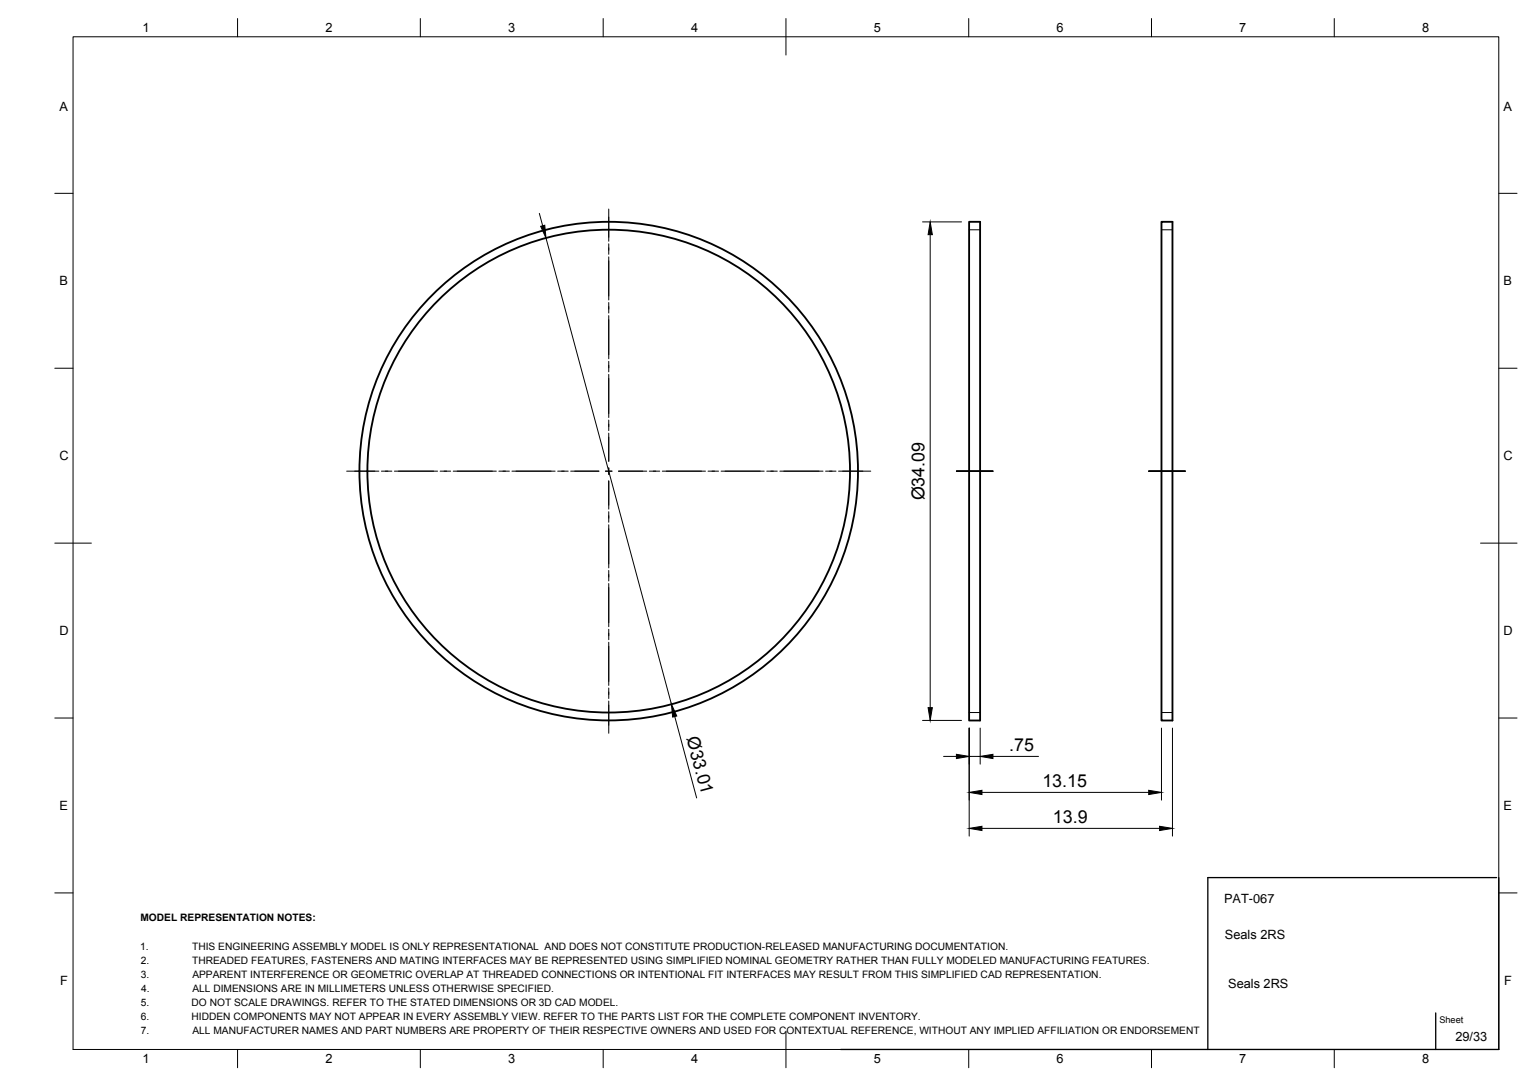
ISO-10303-21;
HEADER;
/* Generated by software containing ST-Developer
 * from STEP Tools, Inc. (www.steptools.com) 
 */

FILE_DESCRIPTION(
/* description */ ('Lifting hook block with sheave'),
/* implementation_level */ '2;1');

FILE_NAME(
/* name */ 'Seals 2RS.step',
/* time_stamp */ '2026-10-28T03:23:54-07:00',
/* author */ (''),
/* organization */ (''),
/* preprocessor_version */ 'ST-DEVELOPER v20.2',
/* originating_system */ 'Autodesk Translation Framework v15.17.0.0',
/* authorisation */ '');

FILE_SCHEMA (('AUTOMOTIVE_DESIGN { 1 0 10303 214 3 1 1 }'));
ENDSEC;

DATA;
#10=MECHANICAL_DESIGN_GEOMETRIC_PRESENTATION_REPRESENTATION('',(#382,#383),#9391);
#315=SHAPE_REPRESENTATION_RELATIONSHIP('SRR','None',#9548,#345);
#345=ADVANCED_BREP_SHAPE_REPRESENTATION('',(#418,#419),#9383);
#382=STYLED_ITEM('',(#9759),#418);
#383=STYLED_ITEM('',(#9759),#419);
#418=MANIFOLD_SOLID_BREP('Body1',#4920);
#419=MANIFOLD_SOLID_BREP('Body2',#4921);
#638=LINE('',#9043,#926);
#639=LINE('',#9048,#927);
#640=LINE('',#9057,#928);
#641=LINE('',#9062,#929);
#926=VECTOR('',#7225,1.70469);
#927=VECTOR('',#7232,1.65031);
#928=VECTOR('',#7243,1.70469);
#929=VECTOR('',#7250,1.65031);
#1089=CYLINDRICAL_SURFACE('',#5798,1.70469);
#1090=CYLINDRICAL_SURFACE('',#5802,1.65031);
#1091=CYLINDRICAL_SURFACE('',#5806,1.70469);
#1092=CYLINDRICAL_SURFACE('',#5810,1.65031);
#1207=FACE_BOUND('',#1842,.T.);
#1208=FACE_BOUND('',#1845,.T.);
#1209=FACE_BOUND('',#1848,.T.);
#1210=FACE_BOUND('',#1851,.T.);
#1452=FACE_OUTER_BOUND('',#1841,.T.);
#1453=FACE_OUTER_BOUND('',#1843,.T.);
#1454=FACE_OUTER_BOUND('',#1844,.T.);
#1455=FACE_OUTER_BOUND('',#1846,.T.);
#1456=FACE_OUTER_BOUND('',#1847,.T.);
#1457=FACE_OUTER_BOUND('',#1849,.T.);
#1458=FACE_OUTER_BOUND('',#1850,.T.);
#1459=FACE_OUTER_BOUND('',#1852,.T.);
#1841=EDGE_LOOP('',(#4222));
#1842=EDGE_LOOP('',(#4223));
#1843=EDGE_LOOP('',(#4224,#4225,#4226,#4227));
#1844=EDGE_LOOP('',(#4228));
#1845=EDGE_LOOP('',(#4229));
#1846=EDGE_LOOP('',(#4230,#4231,#4232,#4233));
#1847=EDGE_LOOP('',(#4234));
#1848=EDGE_LOOP('',(#4235));
#1849=EDGE_LOOP('',(#4236,#4237,#4238,#4239));
#1850=EDGE_LOOP('',(#4240));
#1851=EDGE_LOOP('',(#4241));
#1852=EDGE_LOOP('',(#4242,#4243,#4244,#4245));
#2167=CIRCLE('',#5796,1.70469);
#2168=CIRCLE('',#5797,1.65031);
#2169=CIRCLE('',#5799,1.70469);
#2170=CIRCLE('',#5801,1.65031);
#2171=CIRCLE('',#5804,1.70469);
#2172=CIRCLE('',#5805,1.65031);
#2173=CIRCLE('',#5807,1.70469);
#2174=CIRCLE('',#5809,1.65031);
#2544=VERTEX_POINT('',#9036);
#2545=VERTEX_POINT('',#9038);
#2546=VERTEX_POINT('',#9041);
#2547=VERTEX_POINT('',#9045);
#2548=VERTEX_POINT('',#9050);
#2549=VERTEX_POINT('',#9052);
#2550=VERTEX_POINT('',#9055);
#2551=VERTEX_POINT('',#9059);
#3115=EDGE_CURVE('',#2544,#2544,#2167,.T.);
#3116=EDGE_CURVE('',#2545,#2545,#2168,.T.);
#3117=EDGE_CURVE('',#2546,#2546,#2169,.T.);
#3118=EDGE_CURVE('',#2546,#2544,#638,.T.);
#3119=EDGE_CURVE('',#2547,#2547,#2170,.T.);
#3120=EDGE_CURVE('',#2547,#2545,#639,.T.);
#3121=EDGE_CURVE('',#2548,#2548,#2171,.T.);
#3122=EDGE_CURVE('',#2549,#2549,#2172,.T.);
#3123=EDGE_CURVE('',#2550,#2550,#2173,.T.);
#3124=EDGE_CURVE('',#2550,#2548,#640,.T.);
#3125=EDGE_CURVE('',#2551,#2551,#2174,.T.);
#3126=EDGE_CURVE('',#2551,#2549,#641,.T.);
#4222=ORIENTED_EDGE('',*,*,#3115,.F.);
#4223=ORIENTED_EDGE('',*,*,#3116,.T.);
#4224=ORIENTED_EDGE('',*,*,#3117,.F.);
#4225=ORIENTED_EDGE('',*,*,#3118,.T.);
#4226=ORIENTED_EDGE('',*,*,#3115,.T.);
#4227=ORIENTED_EDGE('',*,*,#3118,.F.);
#4228=ORIENTED_EDGE('',*,*,#3117,.T.);
#4229=ORIENTED_EDGE('',*,*,#3119,.F.);
#4230=ORIENTED_EDGE('',*,*,#3119,.T.);
#4231=ORIENTED_EDGE('',*,*,#3120,.T.);
#4232=ORIENTED_EDGE('',*,*,#3116,.F.);
#4233=ORIENTED_EDGE('',*,*,#3120,.F.);
#4234=ORIENTED_EDGE('',*,*,#3121,.F.);
#4235=ORIENTED_EDGE('',*,*,#3122,.T.);
#4236=ORIENTED_EDGE('',*,*,#3123,.F.);
#4237=ORIENTED_EDGE('',*,*,#3124,.T.);
#4238=ORIENTED_EDGE('',*,*,#3121,.T.);
#4239=ORIENTED_EDGE('',*,*,#3124,.F.);
#4240=ORIENTED_EDGE('',*,*,#3123,.T.);
#4241=ORIENTED_EDGE('',*,*,#3125,.F.);
#4242=ORIENTED_EDGE('',*,*,#3125,.T.);
#4243=ORIENTED_EDGE('',*,*,#3126,.T.);
#4244=ORIENTED_EDGE('',*,*,#3122,.F.);
#4245=ORIENTED_EDGE('',*,*,#3126,.F.);
#4560=PLANE('',#5795);
#4561=PLANE('',#5800);
#4562=PLANE('',#5803);
#4563=PLANE('',#5808);
#4828=ADVANCED_FACE('',(#1452,#1207),#4560,.T.);
#4829=ADVANCED_FACE('',(#1453),#1089,.T.);
#4830=ADVANCED_FACE('',(#1454,#1208),#4561,.T.);
#4831=ADVANCED_FACE('',(#1455),#1090,.F.);
#4832=ADVANCED_FACE('',(#1456,#1209),#4562,.T.);
#4833=ADVANCED_FACE('',(#1457),#1091,.T.);
#4834=ADVANCED_FACE('',(#1458,#1210),#4563,.T.);
#4835=ADVANCED_FACE('',(#1459),#1092,.F.);
#4920=CLOSED_SHELL('',(#4828,#4829,#4830,#4831));
#4921=CLOSED_SHELL('',(#4832,#4833,#4834,#4835));
#5794=AXIS2_PLACEMENT_3D('',#9034,#7213,#7214);
#5795=AXIS2_PLACEMENT_3D('',#9035,#7215,#7216);
#5796=AXIS2_PLACEMENT_3D('',#9037,#7217,#7218);
#5797=AXIS2_PLACEMENT_3D('',#9039,#7219,#7220);
#5798=AXIS2_PLACEMENT_3D('',#9040,#7221,#7222);
#5799=AXIS2_PLACEMENT_3D('',#9042,#7223,#7224);
#5800=AXIS2_PLACEMENT_3D('',#9044,#7226,#7227);
#5801=AXIS2_PLACEMENT_3D('',#9046,#7228,#7229);
#5802=AXIS2_PLACEMENT_3D('',#9047,#7230,#7231);
#5803=AXIS2_PLACEMENT_3D('',#9049,#7233,#7234);
#5804=AXIS2_PLACEMENT_3D('',#9051,#7235,#7236);
#5805=AXIS2_PLACEMENT_3D('',#9053,#7237,#7238);
#5806=AXIS2_PLACEMENT_3D('',#9054,#7239,#7240);
#5807=AXIS2_PLACEMENT_3D('',#9056,#7241,#7242);
#5808=AXIS2_PLACEMENT_3D('',#9058,#7244,#7245);
#5809=AXIS2_PLACEMENT_3D('',#9060,#7246,#7247);
#5810=AXIS2_PLACEMENT_3D('',#9061,#7248,#7249);
#7213=DIRECTION('axis',(0.,0.,1.));
#7214=DIRECTION('refdir',(1.,0.,0.));
#7215=DIRECTION('center_axis',(0.,1.,0.));
#7216=DIRECTION('ref_axis',(0.,0.,1.));
#7217=DIRECTION('center_axis',(0.,-1.,0.));
#7218=DIRECTION('ref_axis',(1.,0.,0.));
#7219=DIRECTION('center_axis',(0.,-1.,0.));
#7220=DIRECTION('ref_axis',(1.,0.,0.));
#7221=DIRECTION('center_axis',(0.,-1.,0.));
#7222=DIRECTION('ref_axis',(1.,0.,0.));
#7223=DIRECTION('center_axis',(0.,-1.,0.));
#7224=DIRECTION('ref_axis',(1.,0.,0.));
#7225=DIRECTION('',(0.,1.,0.));
#7226=DIRECTION('center_axis',(0.,-1.,0.));
#7227=DIRECTION('ref_axis',(0.,0.,-1.));
#7228=DIRECTION('center_axis',(0.,-1.,0.));
#7229=DIRECTION('ref_axis',(1.,0.,0.));
#7230=DIRECTION('center_axis',(0.,-1.,0.));
#7231=DIRECTION('ref_axis',(1.,0.,0.));
#7232=DIRECTION('',(0.,1.,0.));
#7233=DIRECTION('center_axis',(0.,1.,0.));
#7234=DIRECTION('ref_axis',(0.,0.,1.));
#7235=DIRECTION('center_axis',(0.,-1.,0.));
#7236=DIRECTION('ref_axis',(1.,0.,0.));
#7237=DIRECTION('center_axis',(0.,-1.,0.));
#7238=DIRECTION('ref_axis',(1.,0.,0.));
#7239=DIRECTION('center_axis',(0.,-1.,0.));
#7240=DIRECTION('ref_axis',(1.,0.,0.));
#7241=DIRECTION('center_axis',(0.,-1.,0.));
#7242=DIRECTION('ref_axis',(1.,0.,0.));
#7243=DIRECTION('',(0.,1.,0.));
#7244=DIRECTION('center_axis',(0.,-1.,0.));
#7245=DIRECTION('ref_axis',(0.,0.,-1.));
#7246=DIRECTION('center_axis',(0.,-1.,0.));
#7247=DIRECTION('ref_axis',(1.,0.,0.));
#7248=DIRECTION('center_axis',(0.,-1.,0.));
#7249=DIRECTION('ref_axis',(1.,0.,0.));
#7250=DIRECTION('',(0.,1.,0.));
#9034=CARTESIAN_POINT('',(0.,0.,0.));
#9035=CARTESIAN_POINT('Origin',(1.70469,0.695,0.));
#9036=CARTESIAN_POINT('',(-1.70469,0.695,-2.0876431520385E-16));
#9037=CARTESIAN_POINT('Origin',(0.,0.695,0.));
#9038=CARTESIAN_POINT('',(-1.65031,0.695,-2.02104685910087E-16));
#9039=CARTESIAN_POINT('Origin',(0.,0.695,0.));
#9040=CARTESIAN_POINT('Origin',(0.,0.6575,0.));
#9041=CARTESIAN_POINT('',(-1.70469,0.62,-2.0876431520385E-16));
#9042=CARTESIAN_POINT('Origin',(0.,0.62,0.));
#9043=CARTESIAN_POINT('',(-1.70469,0.6575,-2.0876431520385E-16));
#9044=CARTESIAN_POINT('Origin',(1.65031,0.62,0.));
#9045=CARTESIAN_POINT('',(-1.65031,0.62,-2.02104685910087E-16));
#9046=CARTESIAN_POINT('Origin',(0.,0.62,0.));
#9047=CARTESIAN_POINT('Origin',(0.,0.6575,0.));
#9048=CARTESIAN_POINT('',(-1.65031,0.6575,-2.02104685910087E-16));
#9049=CARTESIAN_POINT('Origin',(1.70469,-0.62,0.));
#9050=CARTESIAN_POINT('',(-1.70469,-0.62,-2.0876431520385E-16));
#9051=CARTESIAN_POINT('Origin',(0.,-0.62,0.));
#9052=CARTESIAN_POINT('',(-1.65031,-0.62,-2.02104685910087E-16));
#9053=CARTESIAN_POINT('Origin',(0.,-0.62,0.));
#9054=CARTESIAN_POINT('Origin',(0.,-0.6575,0.));
#9055=CARTESIAN_POINT('',(-1.70469,-0.695,-2.0876431520385E-16));
#9056=CARTESIAN_POINT('Origin',(0.,-0.695,0.));
#9057=CARTESIAN_POINT('',(-1.70469,-0.6575,-2.0876431520385E-16));
#9058=CARTESIAN_POINT('Origin',(1.65031,-0.695,0.));
#9059=CARTESIAN_POINT('',(-1.65031,-0.695,-2.02104685910087E-16));
#9060=CARTESIAN_POINT('Origin',(0.,-0.695,0.));
#9061=CARTESIAN_POINT('Origin',(0.,-0.6575,0.));
#9062=CARTESIAN_POINT('',(-1.65031,-0.6575,-2.02104685910087E-16));
#9346=UNCERTAINTY_MEASURE_WITH_UNIT(LENGTH_MEASURE(0.001),#9392,
'DISTANCE_ACCURACY_VALUE',
'Maximum model space distance between geometric entities at asserted c
onnectivities');
#9354=UNCERTAINTY_MEASURE_WITH_UNIT(LENGTH_MEASURE(0.001),#9392,
'DISTANCE_ACCURACY_VALUE',
'Maximum model space distance between geometric entities at asserted c
onnectivities');
#9383=(
GEOMETRIC_REPRESENTATION_CONTEXT(3)
GLOBAL_UNCERTAINTY_ASSIGNED_CONTEXT((#9346))
GLOBAL_UNIT_ASSIGNED_CONTEXT((#9392,#9394,#9395))
REPRESENTATION_CONTEXT('','3D')
);
#9391=(
GEOMETRIC_REPRESENTATION_CONTEXT(3)
GLOBAL_UNCERTAINTY_ASSIGNED_CONTEXT((#9354))
GLOBAL_UNIT_ASSIGNED_CONTEXT((#9392,#9394,#9395))
REPRESENTATION_CONTEXT('','3D')
);
#9392=(
LENGTH_UNIT()
NAMED_UNIT(*)
SI_UNIT(.CENTI.,.METRE.)
);
#9394=(
NAMED_UNIT(*)
PLANE_ANGLE_UNIT()
SI_UNIT($,.RADIAN.)
);
#9395=(
NAMED_UNIT(*)
SI_UNIT($,.STERADIAN.)
SOLID_ANGLE_UNIT()
);
#9424=SHAPE_DEFINITION_REPRESENTATION(#9485,#9548);
#9485=PRODUCT_DEFINITION_SHAPE('',$,#9585);
#9548=SHAPE_REPRESENTATION('',(#5794),#9383);
#9556=PRODUCT_DEFINITION_CONTEXT('part definition',#9666,'design');
#9585=PRODUCT_DEFINITION('Seals 2RS','Seals 2RS',#9621,#9556);
#9621=PRODUCT_DEFINITION_FORMATION('',$,#9696);
#9666=APPLICATION_CONTEXT(
'Core Data for Automotive Mechanical Design Process');
#9667=PRODUCT_CONTEXT('part definition',#9666,'mechanical');
#9696=PRODUCT('Seals 2RS','Seals 2RS','Seals 2RS',(#9667));
#9753=COLOUR_RGB('Grey',0.48,0.52,0.57);
#9754=FILL_AREA_STYLE_COLOUR('',#9753);
#9755=FILL_AREA_STYLE('',(#9754));
#9756=SURFACE_STYLE_FILL_AREA(#9755);
#9757=SURFACE_SIDE_STYLE('',(#9756));
#9758=SURFACE_STYLE_USAGE(.BOTH.,#9757);
#9759=PRESENTATION_STYLE_ASSIGNMENT((#9758));
ENDSEC;
END-ISO-10303-21;
